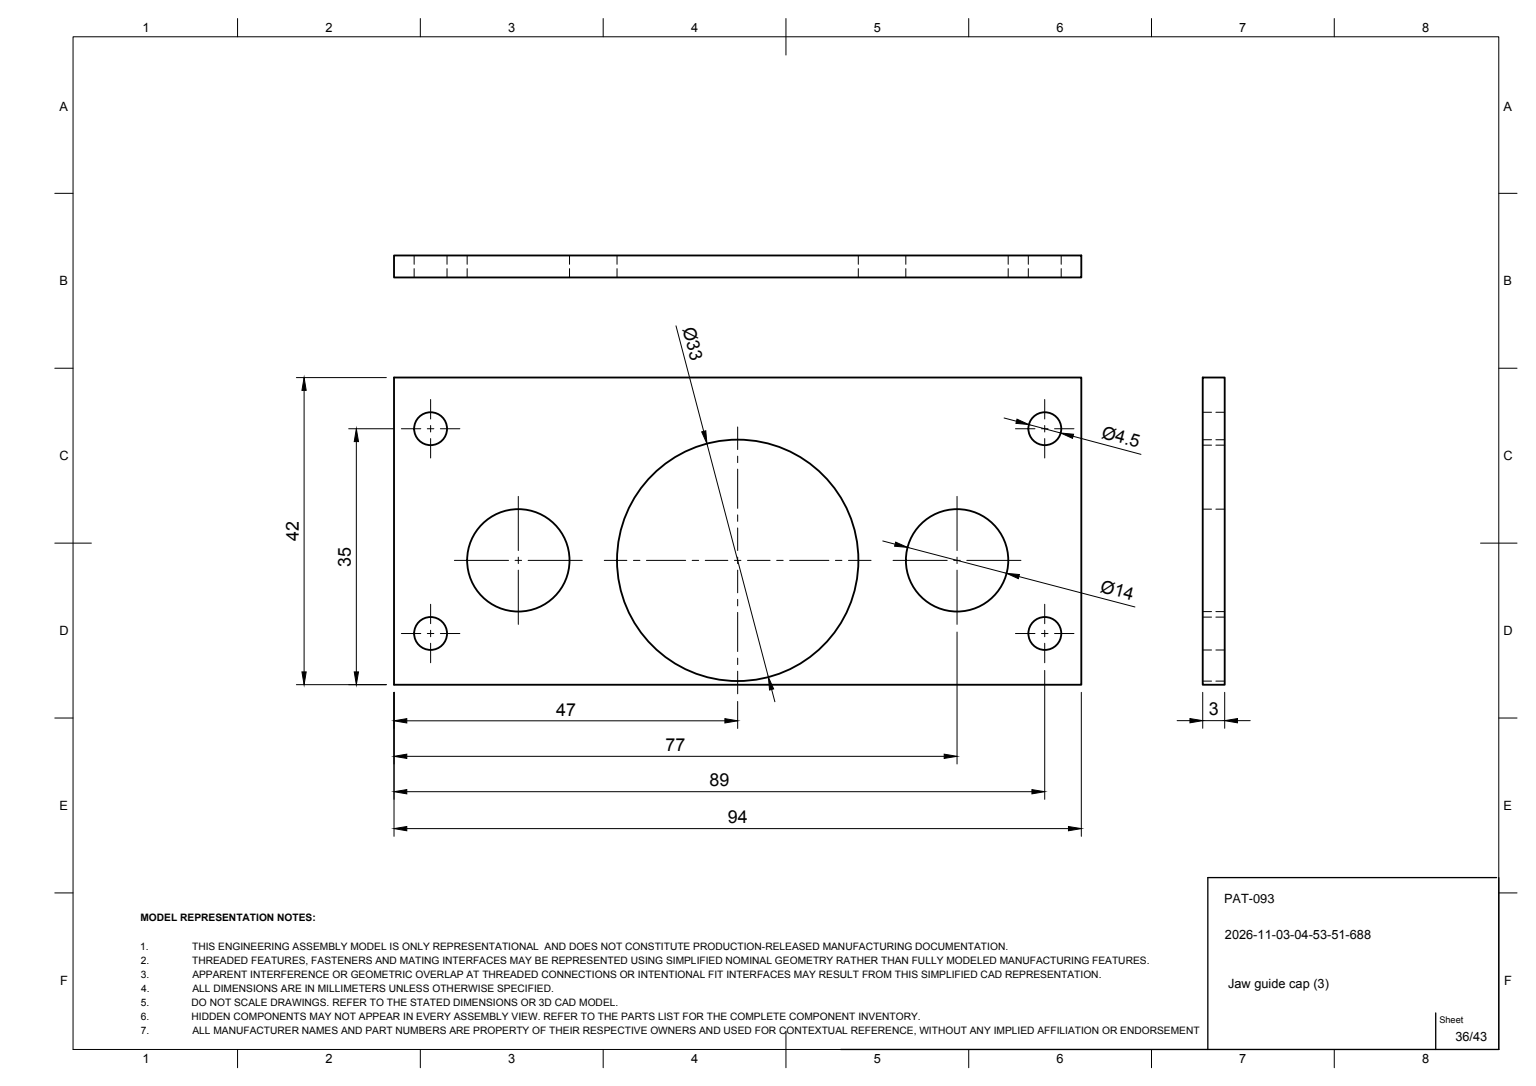
ISO-10303-21;
HEADER;
/* Generated by software containing ST-Developer
 * from STEP Tools, Inc. (www.steptools.com) 
 */

FILE_DESCRIPTION(
/* description */ ('Self-centering screw clamp'),
/* implementation_level */ '2;1');

FILE_NAME(
/* name */ 'Jaw guide cap (3).step',
/* time_stamp */ '2026-10-28T03:25:31-07:00',
/* author */ (''),
/* organization */ (''),
/* preprocessor_version */ 'ST-DEVELOPER v20.2',
/* originating_system */ 'Autodesk Translation Framework v15.17.0.0',
/* authorisation */ '');

FILE_SCHEMA (('AUTOMOTIVE_DESIGN { 1 0 10303 214 3 1 1 }'));
ENDSEC;

DATA;
#10=MECHANICAL_DESIGN_GEOMETRIC_PRESENTATION_REPRESENTATION('',(#657),#16799);
#568=SHAPE_REPRESENTATION_RELATIONSHIP('SRR','None',#17044,#609);
#609=ADVANCED_BREP_SHAPE_REPRESENTATION('',(#705),#16782);
#657=STYLED_ITEM('',(#17312),#705);
#705=MANIFOLD_SOLID_BREP('Body1',#9108);
#950=FACE_BOUND('',#2364,.T.);
#951=FACE_BOUND('',#2365,.T.);
#952=FACE_BOUND('',#2366,.T.);
#953=FACE_BOUND('',#2367,.T.);
#954=FACE_BOUND('',#2368,.T.);
#955=FACE_BOUND('',#2369,.T.);
#956=FACE_BOUND('',#2370,.T.);
#957=FACE_BOUND('',#2373,.T.);
#958=FACE_BOUND('',#2374,.T.);
#959=FACE_BOUND('',#2375,.T.);
#960=FACE_BOUND('',#2376,.T.);
#961=FACE_BOUND('',#2377,.T.);
#962=FACE_BOUND('',#2378,.T.);
#963=FACE_BOUND('',#2379,.T.);
#1179=PLANE('',#10358);
#1180=PLANE('',#10359);
#1181=PLANE('',#10360);
#1182=PLANE('',#10361);
#1183=PLANE('',#10362);
#1184=PLANE('',#10363);
#1619=FACE_OUTER_BOUND('',#2355,.T.);
#1620=FACE_OUTER_BOUND('',#2356,.T.);
#1621=FACE_OUTER_BOUND('',#2357,.T.);
#1622=FACE_OUTER_BOUND('',#2358,.T.);
#1623=FACE_OUTER_BOUND('',#2359,.T.);
#1624=FACE_OUTER_BOUND('',#2360,.T.);
#1625=FACE_OUTER_BOUND('',#2361,.T.);
#1626=FACE_OUTER_BOUND('',#2362,.T.);
#1627=FACE_OUTER_BOUND('',#2363,.T.);
#1628=FACE_OUTER_BOUND('',#2371,.T.);
#1629=FACE_OUTER_BOUND('',#2372,.T.);
#1630=FACE_OUTER_BOUND('',#2380,.T.);
#1631=FACE_OUTER_BOUND('',#2381,.T.);
#2355=EDGE_LOOP('',(#7719,#7720,#7721,#7722));
#2356=EDGE_LOOP('',(#7723,#7724,#7725,#7726));
#2357=EDGE_LOOP('',(#7727,#7728,#7729,#7730));
#2358=EDGE_LOOP('',(#7731,#7732,#7733,#7734));
#2359=EDGE_LOOP('',(#7735,#7736,#7737,#7738));
#2360=EDGE_LOOP('',(#7739,#7740,#7741,#7742));
#2361=EDGE_LOOP('',(#7743,#7744,#7745,#7746));
#2362=EDGE_LOOP('',(#7747,#7748,#7749,#7750));
#2363=EDGE_LOOP('',(#7751,#7752,#7753,#7754));
#2364=EDGE_LOOP('',(#7755));
#2365=EDGE_LOOP('',(#7756));
#2366=EDGE_LOOP('',(#7757));
#2367=EDGE_LOOP('',(#7758));
#2368=EDGE_LOOP('',(#7759));
#2369=EDGE_LOOP('',(#7760));
#2370=EDGE_LOOP('',(#7761));
#2371=EDGE_LOOP('',(#7762,#7763,#7764,#7765));
#2372=EDGE_LOOP('',(#7766,#7767,#7768,#7769));
#2373=EDGE_LOOP('',(#7770));
#2374=EDGE_LOOP('',(#7771));
#2375=EDGE_LOOP('',(#7772));
#2376=EDGE_LOOP('',(#7773));
#2377=EDGE_LOOP('',(#7774));
#2378=EDGE_LOOP('',(#7775));
#2379=EDGE_LOOP('',(#7776));
#2380=EDGE_LOOP('',(#7777,#7778,#7779,#7780));
#2381=EDGE_LOOP('',(#7781,#7782,#7783,#7784));
#2978=LINE('',#15778,#3551);
#2979=LINE('',#15784,#3552);
#2980=LINE('',#15790,#3553);
#2981=LINE('',#15796,#3554);
#2982=LINE('',#15802,#3555);
#2983=LINE('',#15808,#3556);
#2984=LINE('',#15814,#3557);
#2985=LINE('',#15819,#3558);
#2986=LINE('',#15821,#3559);
#2987=LINE('',#15823,#3560);
#2988=LINE('',#15824,#3561);
#2989=LINE('',#15827,#3562);
#2990=LINE('',#15829,#3563);
#2991=LINE('',#15830,#3564);
#2992=LINE('',#15833,#3565);
#2993=LINE('',#15835,#3566);
#2994=LINE('',#15836,#3567);
#2995=LINE('',#15838,#3568);
#2996=LINE('',#15839,#3569);
#3551=VECTOR('',#12677,0.225);
#3552=VECTOR('',#12684,0.225);
#3553=VECTOR('',#12691,0.225);
#3554=VECTOR('',#12698,0.225);
#3555=VECTOR('',#12705,1.65);
#3556=VECTOR('',#12712,0.7);
#3557=VECTOR('',#12719,0.7);
#3558=VECTOR('',#12724,1.);
#3559=VECTOR('',#12725,1.);
#3560=VECTOR('',#12726,1.);
#3561=VECTOR('',#12727,1.);
#3562=VECTOR('',#12730,1.);
#3563=VECTOR('',#12731,1.);
#3564=VECTOR('',#12732,1.);
#3565=VECTOR('',#12735,1.);
#3566=VECTOR('',#12736,1.);
#3567=VECTOR('',#12737,1.);
#3568=VECTOR('',#12740,1.);
#3569=VECTOR('',#12741,1.);
#4100=CIRCLE('',#10338,0.225);
#4101=CIRCLE('',#10339,0.225);
#4102=CIRCLE('',#10341,0.225);
#4103=CIRCLE('',#10342,0.225);
#4104=CIRCLE('',#10344,0.225);
#4105=CIRCLE('',#10345,0.225);
#4106=CIRCLE('',#10347,0.225);
#4107=CIRCLE('',#10348,0.225);
#4108=CIRCLE('',#10350,1.65);
#4109=CIRCLE('',#10351,1.65);
#4110=CIRCLE('',#10353,0.7);
#4111=CIRCLE('',#10354,0.7);
#4112=CIRCLE('',#10356,0.7);
#4113=CIRCLE('',#10357,0.7);
#4767=VERTEX_POINT('',#15775);
#4768=VERTEX_POINT('',#15777);
#4769=VERTEX_POINT('',#15781);
#4770=VERTEX_POINT('',#15783);
#4771=VERTEX_POINT('',#15787);
#4772=VERTEX_POINT('',#15789);
#4773=VERTEX_POINT('',#15793);
#4774=VERTEX_POINT('',#15795);
#4775=VERTEX_POINT('',#15799);
#4776=VERTEX_POINT('',#15801);
#4777=VERTEX_POINT('',#15805);
#4778=VERTEX_POINT('',#15807);
#4779=VERTEX_POINT('',#15811);
#4780=VERTEX_POINT('',#15813);
#4781=VERTEX_POINT('',#15817);
#4782=VERTEX_POINT('',#15818);
#4783=VERTEX_POINT('',#15820);
#4784=VERTEX_POINT('',#15822);
#4785=VERTEX_POINT('',#15826);
#4786=VERTEX_POINT('',#15828);
#4787=VERTEX_POINT('',#15832);
#4788=VERTEX_POINT('',#15834);
#5784=EDGE_CURVE('',#4767,#4767,#4100,.T.);
#5785=EDGE_CURVE('',#4767,#4768,#2978,.T.);
#5786=EDGE_CURVE('',#4768,#4768,#4101,.T.);
#5787=EDGE_CURVE('',#4769,#4769,#4102,.T.);
#5788=EDGE_CURVE('',#4769,#4770,#2979,.T.);
#5789=EDGE_CURVE('',#4770,#4770,#4103,.T.);
#5790=EDGE_CURVE('',#4771,#4771,#4104,.T.);
#5791=EDGE_CURVE('',#4771,#4772,#2980,.T.);
#5792=EDGE_CURVE('',#4772,#4772,#4105,.T.);
#5793=EDGE_CURVE('',#4773,#4773,#4106,.T.);
#5794=EDGE_CURVE('',#4773,#4774,#2981,.T.);
#5795=EDGE_CURVE('',#4774,#4774,#4107,.T.);
#5796=EDGE_CURVE('',#4775,#4775,#4108,.T.);
#5797=EDGE_CURVE('',#4775,#4776,#2982,.T.);
#5798=EDGE_CURVE('',#4776,#4776,#4109,.T.);
#5799=EDGE_CURVE('',#4777,#4777,#4110,.T.);
#5800=EDGE_CURVE('',#4777,#4778,#2983,.T.);
#5801=EDGE_CURVE('',#4778,#4778,#4111,.T.);
#5802=EDGE_CURVE('',#4779,#4779,#4112,.T.);
#5803=EDGE_CURVE('',#4779,#4780,#2984,.T.);
#5804=EDGE_CURVE('',#4780,#4780,#4113,.T.);
#5805=EDGE_CURVE('',#4781,#4782,#2985,.T.);
#5806=EDGE_CURVE('',#4782,#4783,#2986,.T.);
#5807=EDGE_CURVE('',#4784,#4783,#2987,.T.);
#5808=EDGE_CURVE('',#4781,#4784,#2988,.T.);
#5809=EDGE_CURVE('',#4785,#4781,#2989,.T.);
#5810=EDGE_CURVE('',#4786,#4784,#2990,.T.);
#5811=EDGE_CURVE('',#4785,#4786,#2991,.T.);
#5812=EDGE_CURVE('',#4787,#4785,#2992,.T.);
#5813=EDGE_CURVE('',#4788,#4786,#2993,.T.);
#5814=EDGE_CURVE('',#4787,#4788,#2994,.T.);
#5815=EDGE_CURVE('',#4782,#4787,#2995,.T.);
#5816=EDGE_CURVE('',#4783,#4788,#2996,.T.);
#7719=ORIENTED_EDGE('',*,*,#5784,.F.);
#7720=ORIENTED_EDGE('',*,*,#5785,.T.);
#7721=ORIENTED_EDGE('',*,*,#5786,.F.);
#7722=ORIENTED_EDGE('',*,*,#5785,.F.);
#7723=ORIENTED_EDGE('',*,*,#5787,.F.);
#7724=ORIENTED_EDGE('',*,*,#5788,.T.);
#7725=ORIENTED_EDGE('',*,*,#5789,.F.);
#7726=ORIENTED_EDGE('',*,*,#5788,.F.);
#7727=ORIENTED_EDGE('',*,*,#5790,.F.);
#7728=ORIENTED_EDGE('',*,*,#5791,.T.);
#7729=ORIENTED_EDGE('',*,*,#5792,.F.);
#7730=ORIENTED_EDGE('',*,*,#5791,.F.);
#7731=ORIENTED_EDGE('',*,*,#5793,.F.);
#7732=ORIENTED_EDGE('',*,*,#5794,.T.);
#7733=ORIENTED_EDGE('',*,*,#5795,.F.);
#7734=ORIENTED_EDGE('',*,*,#5794,.F.);
#7735=ORIENTED_EDGE('',*,*,#5796,.F.);
#7736=ORIENTED_EDGE('',*,*,#5797,.T.);
#7737=ORIENTED_EDGE('',*,*,#5798,.F.);
#7738=ORIENTED_EDGE('',*,*,#5797,.F.);
#7739=ORIENTED_EDGE('',*,*,#5799,.F.);
#7740=ORIENTED_EDGE('',*,*,#5800,.T.);
#7741=ORIENTED_EDGE('',*,*,#5801,.F.);
#7742=ORIENTED_EDGE('',*,*,#5800,.F.);
#7743=ORIENTED_EDGE('',*,*,#5802,.F.);
#7744=ORIENTED_EDGE('',*,*,#5803,.T.);
#7745=ORIENTED_EDGE('',*,*,#5804,.F.);
#7746=ORIENTED_EDGE('',*,*,#5803,.F.);
#7747=ORIENTED_EDGE('',*,*,#5805,.T.);
#7748=ORIENTED_EDGE('',*,*,#5806,.T.);
#7749=ORIENTED_EDGE('',*,*,#5807,.F.);
#7750=ORIENTED_EDGE('',*,*,#5808,.F.);
#7751=ORIENTED_EDGE('',*,*,#5809,.T.);
#7752=ORIENTED_EDGE('',*,*,#5808,.T.);
#7753=ORIENTED_EDGE('',*,*,#5810,.F.);
#7754=ORIENTED_EDGE('',*,*,#5811,.F.);
#7755=ORIENTED_EDGE('',*,*,#5804,.T.);
#7756=ORIENTED_EDGE('',*,*,#5801,.T.);
#7757=ORIENTED_EDGE('',*,*,#5798,.T.);
#7758=ORIENTED_EDGE('',*,*,#5795,.T.);
#7759=ORIENTED_EDGE('',*,*,#5792,.T.);
#7760=ORIENTED_EDGE('',*,*,#5789,.T.);
#7761=ORIENTED_EDGE('',*,*,#5786,.T.);
#7762=ORIENTED_EDGE('',*,*,#5812,.T.);
#7763=ORIENTED_EDGE('',*,*,#5811,.T.);
#7764=ORIENTED_EDGE('',*,*,#5813,.F.);
#7765=ORIENTED_EDGE('',*,*,#5814,.F.);
#7766=ORIENTED_EDGE('',*,*,#5815,.T.);
#7767=ORIENTED_EDGE('',*,*,#5814,.T.);
#7768=ORIENTED_EDGE('',*,*,#5816,.F.);
#7769=ORIENTED_EDGE('',*,*,#5806,.F.);
#7770=ORIENTED_EDGE('',*,*,#5802,.T.);
#7771=ORIENTED_EDGE('',*,*,#5799,.T.);
#7772=ORIENTED_EDGE('',*,*,#5796,.T.);
#7773=ORIENTED_EDGE('',*,*,#5793,.T.);
#7774=ORIENTED_EDGE('',*,*,#5790,.T.);
#7775=ORIENTED_EDGE('',*,*,#5787,.T.);
#7776=ORIENTED_EDGE('',*,*,#5784,.T.);
#7777=ORIENTED_EDGE('',*,*,#5816,.T.);
#7778=ORIENTED_EDGE('',*,*,#5813,.T.);
#7779=ORIENTED_EDGE('',*,*,#5810,.T.);
#7780=ORIENTED_EDGE('',*,*,#5807,.T.);
#7781=ORIENTED_EDGE('',*,*,#5815,.F.);
#7782=ORIENTED_EDGE('',*,*,#5805,.F.);
#7783=ORIENTED_EDGE('',*,*,#5809,.F.);
#7784=ORIENTED_EDGE('',*,*,#5812,.F.);
#8516=CYLINDRICAL_SURFACE('',#10337,0.225);
#8517=CYLINDRICAL_SURFACE('',#10340,0.225);
#8518=CYLINDRICAL_SURFACE('',#10343,0.225);
#8519=CYLINDRICAL_SURFACE('',#10346,0.225);
#8520=CYLINDRICAL_SURFACE('',#10349,1.65);
#8521=CYLINDRICAL_SURFACE('',#10352,0.7);
#8522=CYLINDRICAL_SURFACE('',#10355,0.7);
#8917=ADVANCED_FACE('',(#1619),#8516,.F.);
#8918=ADVANCED_FACE('',(#1620),#8517,.F.);
#8919=ADVANCED_FACE('',(#1621),#8518,.F.);
#8920=ADVANCED_FACE('',(#1622),#8519,.F.);
#8921=ADVANCED_FACE('',(#1623),#8520,.F.);
#8922=ADVANCED_FACE('',(#1624),#8521,.F.);
#8923=ADVANCED_FACE('',(#1625),#8522,.F.);
#8924=ADVANCED_FACE('',(#1626),#1179,.T.);
#8925=ADVANCED_FACE('',(#1627,#950,#951,#952,#953,#954,#955,#956),#1180,
 .T.);
#8926=ADVANCED_FACE('',(#1628),#1181,.T.);
#8927=ADVANCED_FACE('',(#1629,#957,#958,#959,#960,#961,#962,#963),#1182,
 .T.);
#8928=ADVANCED_FACE('',(#1630),#1183,.T.);
#8929=ADVANCED_FACE('',(#1631),#1184,.F.);
#9108=CLOSED_SHELL('',(#8917,#8918,#8919,#8920,#8921,#8922,#8923,#8924,
#8925,#8926,#8927,#8928,#8929));
#10336=AXIS2_PLACEMENT_3D('',#15773,#12671,#12672);
#10337=AXIS2_PLACEMENT_3D('',#15774,#12673,#12674);
#10338=AXIS2_PLACEMENT_3D('',#15776,#12675,#12676);
#10339=AXIS2_PLACEMENT_3D('',#15779,#12678,#12679);
#10340=AXIS2_PLACEMENT_3D('',#15780,#12680,#12681);
#10341=AXIS2_PLACEMENT_3D('',#15782,#12682,#12683);
#10342=AXIS2_PLACEMENT_3D('',#15785,#12685,#12686);
#10343=AXIS2_PLACEMENT_3D('',#15786,#12687,#12688);
#10344=AXIS2_PLACEMENT_3D('',#15788,#12689,#12690);
#10345=AXIS2_PLACEMENT_3D('',#15791,#12692,#12693);
#10346=AXIS2_PLACEMENT_3D('',#15792,#12694,#12695);
#10347=AXIS2_PLACEMENT_3D('',#15794,#12696,#12697);
#10348=AXIS2_PLACEMENT_3D('',#15797,#12699,#12700);
#10349=AXIS2_PLACEMENT_3D('',#15798,#12701,#12702);
#10350=AXIS2_PLACEMENT_3D('',#15800,#12703,#12704);
#10351=AXIS2_PLACEMENT_3D('',#15803,#12706,#12707);
#10352=AXIS2_PLACEMENT_3D('',#15804,#12708,#12709);
#10353=AXIS2_PLACEMENT_3D('',#15806,#12710,#12711);
#10354=AXIS2_PLACEMENT_3D('',#15809,#12713,#12714);
#10355=AXIS2_PLACEMENT_3D('',#15810,#12715,#12716);
#10356=AXIS2_PLACEMENT_3D('',#15812,#12717,#12718);
#10357=AXIS2_PLACEMENT_3D('',#15815,#12720,#12721);
#10358=AXIS2_PLACEMENT_3D('',#15816,#12722,#12723);
#10359=AXIS2_PLACEMENT_3D('',#15825,#12728,#12729);
#10360=AXIS2_PLACEMENT_3D('',#15831,#12733,#12734);
#10361=AXIS2_PLACEMENT_3D('',#15837,#12738,#12739);
#10362=AXIS2_PLACEMENT_3D('',#15840,#12742,#12743);
#10363=AXIS2_PLACEMENT_3D('',#15841,#12744,#12745);
#12671=DIRECTION('axis',(0.,0.,1.));
#12672=DIRECTION('refdir',(1.,0.,0.));
#12673=DIRECTION('center_axis',(1.,0.,0.));
#12674=DIRECTION('ref_axis',(0.,0.,-1.));
#12675=DIRECTION('center_axis',(1.,0.,0.));
#12676=DIRECTION('ref_axis',(0.,0.,-1.));
#12677=DIRECTION('',(1.,0.,0.));
#12678=DIRECTION('center_axis',(-1.,0.,0.));
#12679=DIRECTION('ref_axis',(0.,0.,-1.));
#12680=DIRECTION('center_axis',(1.,0.,0.));
#12681=DIRECTION('ref_axis',(0.,0.,-1.));
#12682=DIRECTION('center_axis',(1.,0.,0.));
#12683=DIRECTION('ref_axis',(0.,0.,-1.));
#12684=DIRECTION('',(1.,0.,0.));
#12685=DIRECTION('center_axis',(-1.,0.,0.));
#12686=DIRECTION('ref_axis',(0.,0.,-1.));
#12687=DIRECTION('center_axis',(1.,0.,0.));
#12688=DIRECTION('ref_axis',(0.,0.,-1.));
#12689=DIRECTION('center_axis',(1.,0.,0.));
#12690=DIRECTION('ref_axis',(0.,0.,-1.));
#12691=DIRECTION('',(1.,0.,0.));
#12692=DIRECTION('center_axis',(-1.,0.,0.));
#12693=DIRECTION('ref_axis',(0.,0.,-1.));
#12694=DIRECTION('center_axis',(1.,0.,0.));
#12695=DIRECTION('ref_axis',(0.,0.,-1.));
#12696=DIRECTION('center_axis',(1.,0.,0.));
#12697=DIRECTION('ref_axis',(0.,0.,-1.));
#12698=DIRECTION('',(1.,0.,0.));
#12699=DIRECTION('center_axis',(-1.,0.,0.));
#12700=DIRECTION('ref_axis',(0.,0.,-1.));
#12701=DIRECTION('center_axis',(1.,0.,0.));
#12702=DIRECTION('ref_axis',(0.,0.,-1.));
#12703=DIRECTION('center_axis',(1.,0.,0.));
#12704=DIRECTION('ref_axis',(0.,0.,-1.));
#12705=DIRECTION('',(1.,0.,0.));
#12706=DIRECTION('center_axis',(-1.,0.,0.));
#12707=DIRECTION('ref_axis',(0.,0.,-1.));
#12708=DIRECTION('center_axis',(1.,0.,0.));
#12709=DIRECTION('ref_axis',(0.,0.,-1.));
#12710=DIRECTION('center_axis',(1.,0.,0.));
#12711=DIRECTION('ref_axis',(0.,0.,-1.));
#12712=DIRECTION('',(1.,0.,0.));
#12713=DIRECTION('center_axis',(-1.,0.,0.));
#12714=DIRECTION('ref_axis',(0.,0.,-1.));
#12715=DIRECTION('center_axis',(1.,0.,0.));
#12716=DIRECTION('ref_axis',(0.,0.,-1.));
#12717=DIRECTION('center_axis',(1.,0.,0.));
#12718=DIRECTION('ref_axis',(0.,0.,-1.));
#12719=DIRECTION('',(1.,0.,0.));
#12720=DIRECTION('center_axis',(-1.,0.,0.));
#12721=DIRECTION('ref_axis',(0.,0.,-1.));
#12722=DIRECTION('center_axis',(0.,1.,0.));
#12723=DIRECTION('ref_axis',(-1.,0.,0.));
#12724=DIRECTION('',(-1.,0.,0.));
#12725=DIRECTION('',(0.,0.,1.));
#12726=DIRECTION('',(-1.,0.,0.));
#12727=DIRECTION('',(0.,0.,1.));
#12728=DIRECTION('center_axis',(1.,0.,0.));
#12729=DIRECTION('ref_axis',(0.,1.,0.));
#12730=DIRECTION('',(0.,1.,0.));
#12731=DIRECTION('',(0.,1.,0.));
#12732=DIRECTION('',(0.,0.,1.));
#12733=DIRECTION('center_axis',(0.,-1.,0.));
#12734=DIRECTION('ref_axis',(1.,0.,0.));
#12735=DIRECTION('',(1.,0.,0.));
#12736=DIRECTION('',(1.,0.,0.));
#12737=DIRECTION('',(0.,0.,1.));
#12738=DIRECTION('center_axis',(-1.,0.,0.));
#12739=DIRECTION('ref_axis',(0.,-1.,0.));
#12740=DIRECTION('',(0.,-1.,0.));
#12741=DIRECTION('',(0.,-1.,0.));
#12742=DIRECTION('center_axis',(0.,0.,1.));
#12743=DIRECTION('ref_axis',(1.,0.,0.));
#12744=DIRECTION('center_axis',(0.,0.,1.));
#12745=DIRECTION('ref_axis',(1.,0.,0.));
#15773=CARTESIAN_POINT('',(0.,0.,0.));
#15774=CARTESIAN_POINT('Origin',(8.4,4.2,3.));
#15775=CARTESIAN_POINT('',(8.5,4.2,3.225));
#15776=CARTESIAN_POINT('Origin',(8.5,4.2,3.));
#15777=CARTESIAN_POINT('',(8.8,4.2,3.225));
#15778=CARTESIAN_POINT('',(8.4,4.2,3.225));
#15779=CARTESIAN_POINT('Origin',(8.8,4.2,3.));
#15780=CARTESIAN_POINT('Origin',(8.4,-4.2,5.8));
#15781=CARTESIAN_POINT('',(8.5,-4.2,6.025));
#15782=CARTESIAN_POINT('Origin',(8.5,-4.2,5.8));
#15783=CARTESIAN_POINT('',(8.8,-4.2,6.025));
#15784=CARTESIAN_POINT('',(8.4,-4.2,6.025));
#15785=CARTESIAN_POINT('Origin',(8.8,-4.2,5.8));
#15786=CARTESIAN_POINT('Origin',(8.4,-4.2,3.));
#15787=CARTESIAN_POINT('',(8.5,-4.2,3.225));
#15788=CARTESIAN_POINT('Origin',(8.5,-4.2,3.));
#15789=CARTESIAN_POINT('',(8.8,-4.2,3.225));
#15790=CARTESIAN_POINT('',(8.4,-4.2,3.225));
#15791=CARTESIAN_POINT('Origin',(8.8,-4.2,3.));
#15792=CARTESIAN_POINT('Origin',(8.4,4.2,5.8));
#15793=CARTESIAN_POINT('',(8.5,4.2,6.025));
#15794=CARTESIAN_POINT('Origin',(8.5,4.2,5.8));
#15795=CARTESIAN_POINT('',(8.8,4.2,6.025));
#15796=CARTESIAN_POINT('',(8.4,4.2,6.025));
#15797=CARTESIAN_POINT('Origin',(8.8,4.2,5.8));
#15798=CARTESIAN_POINT('Origin',(8.4,0.,4.));
#15799=CARTESIAN_POINT('',(8.5,-2.02066721859313E-16,5.65));
#15800=CARTESIAN_POINT('Origin',(8.5,0.,4.));
#15801=CARTESIAN_POINT('',(8.8,2.02066721859313E-16,5.65));
#15802=CARTESIAN_POINT('',(8.4,-2.02066721859313E-16,5.65));
#15803=CARTESIAN_POINT('Origin',(8.8,0.,4.));
#15804=CARTESIAN_POINT('Origin',(8.4,-3.,4.));
#15805=CARTESIAN_POINT('',(8.5,-3.,4.7));
#15806=CARTESIAN_POINT('Origin',(8.5,-3.,4.));
#15807=CARTESIAN_POINT('',(8.8,-3.,4.7));
#15808=CARTESIAN_POINT('',(8.4,-3.,4.7));
#15809=CARTESIAN_POINT('Origin',(8.8,-3.,4.));
#15810=CARTESIAN_POINT('Origin',(8.4,3.,4.));
#15811=CARTESIAN_POINT('',(8.5,3.,4.7));
#15812=CARTESIAN_POINT('Origin',(8.5,3.,4.));
#15813=CARTESIAN_POINT('',(8.8,3.,4.7));
#15814=CARTESIAN_POINT('',(8.4,3.,4.7));
#15815=CARTESIAN_POINT('Origin',(8.8,3.,4.));
#15816=CARTESIAN_POINT('Origin',(8.8,4.7,2.3));
#15817=CARTESIAN_POINT('',(8.8,4.7,2.3));
#15818=CARTESIAN_POINT('',(8.5,4.7,2.3));
#15819=CARTESIAN_POINT('',(8.8,4.7,2.3));
#15820=CARTESIAN_POINT('',(8.5,4.7,6.5));
#15821=CARTESIAN_POINT('',(8.5,4.7,2.3));
#15822=CARTESIAN_POINT('',(8.8,4.7,6.5));
#15823=CARTESIAN_POINT('',(8.8,4.7,6.5));
#15824=CARTESIAN_POINT('',(8.8,4.7,2.3));
#15825=CARTESIAN_POINT('Origin',(8.8,-4.7,2.3));
#15826=CARTESIAN_POINT('',(8.8,-4.7,2.3));
#15827=CARTESIAN_POINT('',(8.8,-4.7,2.3));
#15828=CARTESIAN_POINT('',(8.8,-4.7,6.5));
#15829=CARTESIAN_POINT('',(8.8,-4.7,6.5));
#15830=CARTESIAN_POINT('',(8.8,-4.7,2.3));
#15831=CARTESIAN_POINT('Origin',(8.5,-4.7,2.3));
#15832=CARTESIAN_POINT('',(8.5,-4.7,2.3));
#15833=CARTESIAN_POINT('',(8.5,-4.7,2.3));
#15834=CARTESIAN_POINT('',(8.5,-4.7,6.5));
#15835=CARTESIAN_POINT('',(8.5,-4.7,6.5));
#15836=CARTESIAN_POINT('',(8.5,-4.7,2.3));
#15837=CARTESIAN_POINT('Origin',(8.5,4.7,2.3));
#15838=CARTESIAN_POINT('',(8.5,4.7,2.3));
#15839=CARTESIAN_POINT('',(8.5,4.7,6.5));
#15840=CARTESIAN_POINT('Origin',(8.65,0.,6.5));
#15841=CARTESIAN_POINT('Origin',(8.65,0.,2.3));
#16733=UNCERTAINTY_MEASURE_WITH_UNIT(LENGTH_MEASURE(0.001),#16800,
'DISTANCE_ACCURACY_VALUE',
'Maximum model space distance between geometric entities at asserted c
onnectivities');
#16750=UNCERTAINTY_MEASURE_WITH_UNIT(LENGTH_MEASURE(0.001),#16800,
'DISTANCE_ACCURACY_VALUE',
'Maximum model space distance between geometric entities at asserted c
onnectivities');
#16782=(
GEOMETRIC_REPRESENTATION_CONTEXT(3)
GLOBAL_UNCERTAINTY_ASSIGNED_CONTEXT((#16733))
GLOBAL_UNIT_ASSIGNED_CONTEXT((#16800,#16802,#16803))
REPRESENTATION_CONTEXT('','3D')
);
#16799=(
GEOMETRIC_REPRESENTATION_CONTEXT(3)
GLOBAL_UNCERTAINTY_ASSIGNED_CONTEXT((#16750))
GLOBAL_UNIT_ASSIGNED_CONTEXT((#16800,#16802,#16803))
REPRESENTATION_CONTEXT('','3D')
);
#16800=(
LENGTH_UNIT()
NAMED_UNIT(*)
SI_UNIT(.CENTI.,.METRE.)
);
#16802=(
NAMED_UNIT(*)
PLANE_ANGLE_UNIT()
SI_UNIT($,.RADIAN.)
);
#16803=(
NAMED_UNIT(*)
SI_UNIT($,.STERADIAN.)
SOLID_ANGLE_UNIT()
);
#16835=SHAPE_DEFINITION_REPRESENTATION(#16888,#17044);
#16888=PRODUCT_DEFINITION_SHAPE('',$,#17093);
#17044=SHAPE_REPRESENTATION('',(#10336),#16782);
#17061=PRODUCT_DEFINITION_CONTEXT('part definition',#17207,'design');
#17093=PRODUCT_DEFINITION('Jaw guide cap (3)','Jaw guide cap (3)',#17141,
#17061);
#17141=PRODUCT_DEFINITION_FORMATION('',$,#17240);
#17207=APPLICATION_CONTEXT(
'Core Data for Automotive Mechanical Design Process');
#17208=PRODUCT_CONTEXT('part definition',#17207,'mechanical');
#17240=PRODUCT('Jaw guide cap (3)','Jaw guide cap (3)','Jaw guide cap (3)',(#17208));
#17306=COLOUR_RGB('Light Blue',0.38,0.62,0.78);
#17307=FILL_AREA_STYLE_COLOUR('',#17306);
#17308=FILL_AREA_STYLE('',(#17307));
#17309=SURFACE_STYLE_FILL_AREA(#17308);
#17310=SURFACE_SIDE_STYLE('',(#17309));
#17311=SURFACE_STYLE_USAGE(.BOTH.,#17310);
#17312=PRESENTATION_STYLE_ASSIGNMENT((#17311));
ENDSEC;
END-ISO-10303-21;
